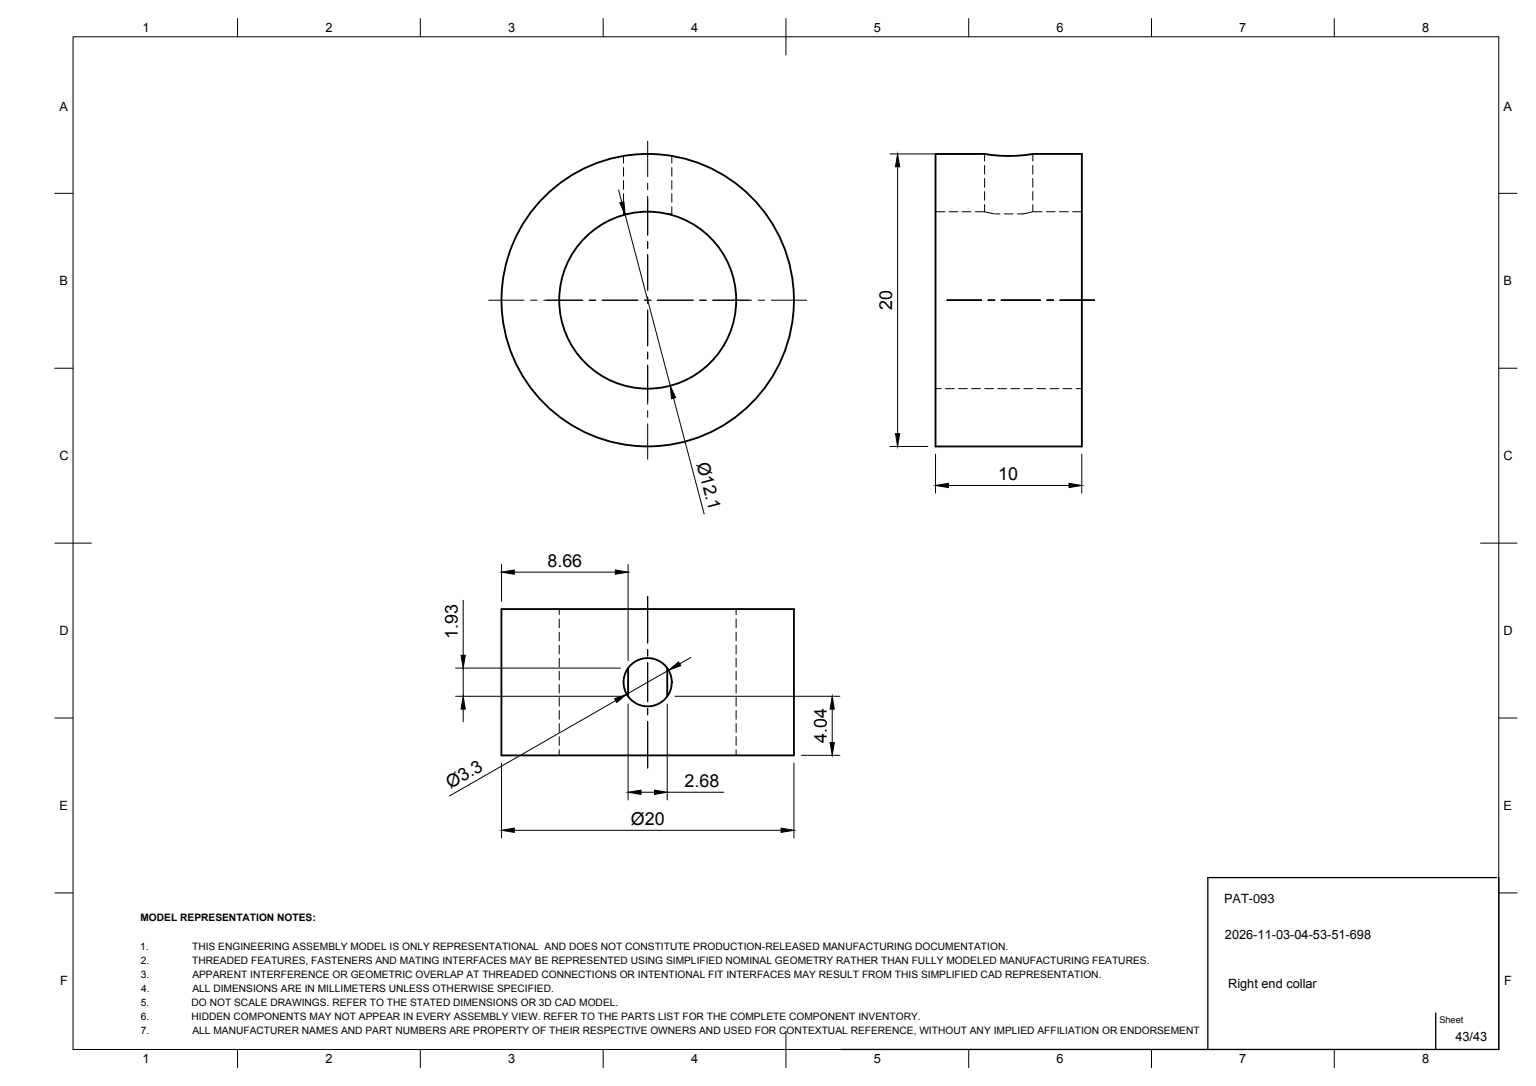
ISO-10303-21;
HEADER;
/* Generated by software containing ST-Developer
 * from STEP Tools, Inc. (www.steptools.com) 
 */

FILE_DESCRIPTION(
/* description */ ('Self-centering screw clamp'),
/* implementation_level */ '2;1');

FILE_NAME(
/* name */ 'Right end collar.step',
/* time_stamp */ '2026-10-28T03:25:31-07:00',
/* author */ (''),
/* organization */ (''),
/* preprocessor_version */ 'ST-DEVELOPER v20.2',
/* originating_system */ 'Autodesk Translation Framework v15.17.0.0',
/* authorisation */ '');

FILE_SCHEMA (('AUTOMOTIVE_DESIGN { 1 0 10303 214 3 1 1 }'));
ENDSEC;

DATA;
#10=MECHANICAL_DESIGN_GEOMETRIC_PRESENTATION_REPRESENTATION('',(#669),#16799);
#535=B_SPLINE_CURVE_WITH_KNOTS('',3,(#16377,#16378,#16379,#16380,#16381,
#16382,#16383,#16384),.UNSPECIFIED.,.F.,.F.,(4,2,2,4),(0.598759573717649,
0.624973342427789,0.687463163426141,0.749952984424493),.UNSPECIFIED.);
#536=B_SPLINE_CURVE_WITH_KNOTS('',3,(#16388,#16389,#16390,#16391,#16392,
#16393,#16394,#16395),.UNSPECIFIED.,.F.,.F.,(4,2,2,4),(0.249984328141498,
0.31247414913985,0.374963970138202,0.401177738848341),.UNSPECIFIED.);
#537=B_SPLINE_CURVE_WITH_KNOTS('',3,(#16396,#16397,#16398,#16399,#16400,
#16401,#16402,#16403),.UNSPECIFIED.,.F.,.F.,(4,2,2,4),(0.0987909174346529,
0.125004686144794,0.187494507143146,0.249984328141498),.UNSPECIFIED.);
#538=B_SPLINE_CURVE_WITH_KNOTS('',3,(#16404,#16405,#16406,#16407,#16408,
#16409,#16410,#16411),.UNSPECIFIED.,.F.,.F.,(4,2,2,4),(0.749952984424493,
0.812442805422846,0.874932626421198,0.901146395131338),.UNSPECIFIED.);
#539=B_SPLINE_CURVE_WITH_KNOTS('',3,(#16415,#16416,#16417,#16418,#16419,
#16420,#16421,#16422,#16423,#16424),.UNSPECIFIED.,.F.,.F.,(4,2,2,2,4),(0.,
0.0622766332261793,0.124553266452359,0.186828302721277,0.249103338990195),
 .UNSPECIFIED.);
#540=B_SPLINE_CURVE_WITH_KNOTS('',3,(#16426,#16427,#16428,#16429,#16430,
#16431,#16432,#16433,#16434,#16435),.UNSPECIFIED.,.F.,.F.,(4,2,2,2,4),(0.747310016970586,
0.809585053239505,0.871860089508423,0.934136722734602,0.996413355960782),
 .UNSPECIFIED.);
#541=B_SPLINE_CURVE_WITH_KNOTS('',3,(#16436,#16437,#16438,#16439,#16440,
#16441,#16442,#16443,#16444,#16445,#16446,#16447,#16448,#16449,#16450,#16451,
#16452,#16453),.UNSPECIFIED.,.F.,.F.,(4,2,2,2,2,2,2,2,4),(0.249103338990195,
0.311378375259114,0.373653411528032,0.435930044754212,0.498206677980391,
0.56048331120657,0.62275994443275,0.685034980701668,0.747310016970586),
 .UNSPECIFIED.);
#580=SHAPE_REPRESENTATION_RELATIONSHIP('SRR','None',#17058,#621);
#621=ADVANCED_BREP_SHAPE_REPRESENTATION('',(#716),#16796);
#669=STYLED_ITEM('',(#17340),#716);
#716=MANIFOLD_SOLID_BREP('Body1',#9121);
#1010=FACE_BOUND('',#2543,.T.);
#1011=FACE_BOUND('',#2545,.T.);
#1249=PLANE('',#10590);
#1250=PLANE('',#10594);
#1251=PLANE('',#10601);
#1252=PLANE('',#10602);
#1741=FACE_OUTER_BOUND('',#2537,.T.);
#1742=FACE_OUTER_BOUND('',#2538,.T.);
#1743=FACE_OUTER_BOUND('',#2539,.T.);
#1744=FACE_OUTER_BOUND('',#2540,.T.);
#1745=FACE_OUTER_BOUND('',#2541,.T.);
#1746=FACE_OUTER_BOUND('',#2542,.T.);
#1747=FACE_OUTER_BOUND('',#2544,.T.);
#2537=EDGE_LOOP('',(#8203,#8204));
#2538=EDGE_LOOP('',(#8205,#8206,#8207,#8208,#8209,#8210,#8211,#8212,#8213,
#8214,#8215));
#2539=EDGE_LOOP('',(#8216,#8217));
#2540=EDGE_LOOP('',(#8218,#8219,#8220,#8221,#8222,#8223,#8224,#8225,#8226,
#8227,#8228,#8229));
#2541=EDGE_LOOP('',(#8230,#8231,#8232,#8233,#8234,#8235,#8236,#8237,#8238));
#2542=EDGE_LOOP('',(#8239));
#2543=EDGE_LOOP('',(#8240));
#2544=EDGE_LOOP('',(#8241));
#2545=EDGE_LOOP('',(#8242));
#3098=LINE('',#16372,#3671);
#3099=LINE('',#16413,#3672);
#3100=LINE('',#16455,#3673);
#3101=LINE('',#16459,#3674);
#3102=LINE('',#16461,#3675);
#3103=LINE('',#16466,#3676);
#3104=LINE('',#16468,#3677);
#3671=VECTOR('',#13301,1.);
#3672=VECTOR('',#13308,0.164999999999999);
#3673=VECTOR('',#13311,1.);
#3674=VECTOR('',#13316,0.605);
#3675=VECTOR('',#13317,0.605);
#3676=VECTOR('',#13324,1.);
#3677=VECTOR('',#13325,1.);
#4215=CIRCLE('',#10591,0.164999999999999);
#4216=CIRCLE('',#10593,0.164999999999999);
#4217=CIRCLE('',#10596,0.605);
#4218=CIRCLE('',#10597,0.605);
#4219=CIRCLE('',#10599,1.);
#4220=CIRCLE('',#10600,1.);
#4927=VERTEX_POINT('',#16370);
#4928=VERTEX_POINT('',#16371);
#4929=VERTEX_POINT('',#16375);
#4930=VERTEX_POINT('',#16376);
#4931=VERTEX_POINT('',#16385);
#4932=VERTEX_POINT('',#16387);
#4933=VERTEX_POINT('',#16412);
#4934=VERTEX_POINT('',#16414);
#4935=VERTEX_POINT('',#16425);
#4936=VERTEX_POINT('',#16457);
#4937=VERTEX_POINT('',#16460);
#4938=VERTEX_POINT('',#16464);
#4939=VERTEX_POINT('',#16467);
#6026=EDGE_CURVE('',#4927,#4928,#3098,.T.);
#6027=EDGE_CURVE('',#4927,#4928,#4215,.T.);
#6028=EDGE_CURVE('',#4929,#4930,#535,.T.);
#6029=EDGE_CURVE('',#4931,#4929,#4216,.T.);
#6030=EDGE_CURVE('',#4932,#4931,#536,.T.);
#6031=EDGE_CURVE('',#4928,#4932,#537,.T.);
#6032=EDGE_CURVE('',#4930,#4927,#538,.T.);
#6033=EDGE_CURVE('',#4930,#4933,#3099,.T.);
#6034=EDGE_CURVE('',#4934,#4933,#539,.T.);
#6035=EDGE_CURVE('',#4935,#4934,#540,.T.);
#6036=EDGE_CURVE('',#4933,#4935,#541,.T.);
#6037=EDGE_CURVE('',#4931,#4929,#3100,.T.);
#6038=EDGE_CURVE('',#4936,#4936,#4217,.T.);
#6039=EDGE_CURVE('',#4936,#4932,#3101,.T.);
#6040=EDGE_CURVE('',#4930,#4937,#3102,.T.);
#6041=EDGE_CURVE('',#4937,#4937,#4218,.T.);
#6042=EDGE_CURVE('',#4938,#4938,#4219,.T.);
#6043=EDGE_CURVE('',#4938,#4935,#3103,.T.);
#6044=EDGE_CURVE('',#4933,#4939,#3104,.T.);
#6045=EDGE_CURVE('',#4939,#4939,#4220,.T.);
#8203=ORIENTED_EDGE('',*,*,#6026,.F.);
#8204=ORIENTED_EDGE('',*,*,#6027,.T.);
#8205=ORIENTED_EDGE('',*,*,#6028,.F.);
#8206=ORIENTED_EDGE('',*,*,#6029,.F.);
#8207=ORIENTED_EDGE('',*,*,#6030,.F.);
#8208=ORIENTED_EDGE('',*,*,#6031,.F.);
#8209=ORIENTED_EDGE('',*,*,#6027,.F.);
#8210=ORIENTED_EDGE('',*,*,#6032,.F.);
#8211=ORIENTED_EDGE('',*,*,#6033,.T.);
#8212=ORIENTED_EDGE('',*,*,#6034,.F.);
#8213=ORIENTED_EDGE('',*,*,#6035,.F.);
#8214=ORIENTED_EDGE('',*,*,#6036,.F.);
#8215=ORIENTED_EDGE('',*,*,#6033,.F.);
#8216=ORIENTED_EDGE('',*,*,#6037,.F.);
#8217=ORIENTED_EDGE('',*,*,#6029,.T.);
#8218=ORIENTED_EDGE('',*,*,#6038,.F.);
#8219=ORIENTED_EDGE('',*,*,#6039,.T.);
#8220=ORIENTED_EDGE('',*,*,#6030,.T.);
#8221=ORIENTED_EDGE('',*,*,#6037,.T.);
#8222=ORIENTED_EDGE('',*,*,#6028,.T.);
#8223=ORIENTED_EDGE('',*,*,#6040,.T.);
#8224=ORIENTED_EDGE('',*,*,#6041,.T.);
#8225=ORIENTED_EDGE('',*,*,#6040,.F.);
#8226=ORIENTED_EDGE('',*,*,#6032,.T.);
#8227=ORIENTED_EDGE('',*,*,#6026,.T.);
#8228=ORIENTED_EDGE('',*,*,#6031,.T.);
#8229=ORIENTED_EDGE('',*,*,#6039,.F.);
#8230=ORIENTED_EDGE('',*,*,#6042,.F.);
#8231=ORIENTED_EDGE('',*,*,#6043,.T.);
#8232=ORIENTED_EDGE('',*,*,#6035,.T.);
#8233=ORIENTED_EDGE('',*,*,#6034,.T.);
#8234=ORIENTED_EDGE('',*,*,#6044,.T.);
#8235=ORIENTED_EDGE('',*,*,#6045,.T.);
#8236=ORIENTED_EDGE('',*,*,#6044,.F.);
#8237=ORIENTED_EDGE('',*,*,#6036,.T.);
#8238=ORIENTED_EDGE('',*,*,#6043,.F.);
#8239=ORIENTED_EDGE('',*,*,#6042,.T.);
#8240=ORIENTED_EDGE('',*,*,#6038,.T.);
#8241=ORIENTED_EDGE('',*,*,#6045,.F.);
#8242=ORIENTED_EDGE('',*,*,#6041,.F.);
#8565=CYLINDRICAL_SURFACE('',#10592,0.164999999999999);
#8566=CYLINDRICAL_SURFACE('',#10595,0.605);
#8567=CYLINDRICAL_SURFACE('',#10598,1.);
#9039=ADVANCED_FACE('',(#1741),#1249,.T.);
#9040=ADVANCED_FACE('',(#1742),#8565,.F.);
#9041=ADVANCED_FACE('',(#1743),#1250,.T.);
#9042=ADVANCED_FACE('',(#1744),#8566,.F.);
#9043=ADVANCED_FACE('',(#1745),#8567,.T.);
#9044=ADVANCED_FACE('',(#1746,#1010),#1251,.T.);
#9045=ADVANCED_FACE('',(#1747,#1011),#1252,.F.);
#9121=CLOSED_SHELL('',(#9039,#9040,#9041,#9042,#9043,#9044,#9045));
#10589=AXIS2_PLACEMENT_3D('',#16368,#13297,#13298);
#10590=AXIS2_PLACEMENT_3D('',#16369,#13299,#13300);
#10591=AXIS2_PLACEMENT_3D('',#16373,#13302,#13303);
#10592=AXIS2_PLACEMENT_3D('',#16374,#13304,#13305);
#10593=AXIS2_PLACEMENT_3D('',#16386,#13306,#13307);
#10594=AXIS2_PLACEMENT_3D('',#16454,#13309,#13310);
#10595=AXIS2_PLACEMENT_3D('',#16456,#13312,#13313);
#10596=AXIS2_PLACEMENT_3D('',#16458,#13314,#13315);
#10597=AXIS2_PLACEMENT_3D('',#16462,#13318,#13319);
#10598=AXIS2_PLACEMENT_3D('',#16463,#13320,#13321);
#10599=AXIS2_PLACEMENT_3D('',#16465,#13322,#13323);
#10600=AXIS2_PLACEMENT_3D('',#16469,#13326,#13327);
#10601=AXIS2_PLACEMENT_3D('',#16470,#13328,#13329);
#10602=AXIS2_PLACEMENT_3D('',#16471,#13330,#13331);
#13297=DIRECTION('axis',(0.,0.,1.));
#13298=DIRECTION('refdir',(1.,0.,0.));
#13299=DIRECTION('center_axis',(0.,0.,1.));
#13300=DIRECTION('ref_axis',(1.,0.,0.));
#13301=DIRECTION('',(1.,0.,0.));
#13302=DIRECTION('center_axis',(0.,0.,1.));
#13303=DIRECTION('ref_axis',(1.,0.,0.));
#13304=DIRECTION('center_axis',(0.,0.,1.));
#13305=DIRECTION('ref_axis',(1.,0.,0.));
#13306=DIRECTION('center_axis',(0.,0.,1.));
#13307=DIRECTION('ref_axis',(1.,0.,0.));
#13308=DIRECTION('',(0.,0.,1.));
#13309=DIRECTION('center_axis',(0.,0.,1.));
#13310=DIRECTION('ref_axis',(1.,0.,0.));
#13311=DIRECTION('',(-1.,0.,0.));
#13312=DIRECTION('center_axis',(1.,0.,0.));
#13313=DIRECTION('ref_axis',(0.,0.,-1.));
#13314=DIRECTION('center_axis',(-1.,0.,0.));
#13315=DIRECTION('ref_axis',(0.,0.,-1.));
#13316=DIRECTION('',(-1.,0.,0.));
#13317=DIRECTION('',(-1.,0.,0.));
#13318=DIRECTION('center_axis',(-1.,0.,0.));
#13319=DIRECTION('ref_axis',(0.,0.,-1.));
#13320=DIRECTION('center_axis',(1.,0.,0.));
#13321=DIRECTION('ref_axis',(0.,0.,-1.));
#13322=DIRECTION('center_axis',(1.,0.,0.));
#13323=DIRECTION('ref_axis',(0.,0.,-1.));
#13324=DIRECTION('',(-1.,0.,0.));
#13325=DIRECTION('',(-1.,0.,0.));
#13326=DIRECTION('center_axis',(1.,0.,0.));
#13327=DIRECTION('ref_axis',(0.,0.,-1.));
#13328=DIRECTION('center_axis',(1.,0.,0.));
#13329=DIRECTION('ref_axis',(0.,0.,-1.));
#13330=DIRECTION('center_axis',(1.,0.,0.));
#13331=DIRECTION('ref_axis',(0.,0.,-1.));
#16368=CARTESIAN_POINT('',(0.,0.,0.));
#16369=CARTESIAN_POINT('Origin',(14.,0.,4.59));
#16370=CARTESIAN_POINT('',(13.9035634923901,-0.133884278389959,4.59));
#16371=CARTESIAN_POINT('',(14.0964365076099,-0.133884278389959,4.59));
#16372=CARTESIAN_POINT('',(13.5,-0.133884278389959,4.59));
#16373=CARTESIAN_POINT('Origin',(14.,0.,4.59));
#16374=CARTESIAN_POINT('Origin',(14.,0.,4.59));
#16375=CARTESIAN_POINT('',(13.9035634923901,0.133884278389959,4.59));
#16376=CARTESIAN_POINT('',(13.835,-8.64311690359451E-17,4.605));
#16377=CARTESIAN_POINT('Ctrl Pts',(13.9035634923901,0.133884278389959,4.59));
#16378=CARTESIAN_POINT('Ctrl Pts',(13.8962316423768,0.128603165341393,4.59119840340611));
#16379=CARTESIAN_POINT('Ctrl Pts',(13.8894472111884,0.122792448979943,4.59244064128815));
#16380=CARTESIAN_POINT('Ctrl Pts',(13.8687385941683,0.10208383195986,4.59651064111414));
#16381=CARTESIAN_POINT('Ctrl Pts',(13.8560565239921,0.0836002135946602,
4.59954409498317));
#16382=CARTESIAN_POINT('Ctrl Pts',(13.8391843843662,0.0429774150042655,
4.60381707438298));
#16383=CARTESIAN_POINT('Ctrl Pts',(13.835,0.0208299403327843,4.605));
#16384=CARTESIAN_POINT('Ctrl Pts',(13.835,1.94289029309402E-16,4.605));
#16385=CARTESIAN_POINT('',(14.0964365076099,0.133884278389959,4.59));
#16386=CARTESIAN_POINT('Origin',(14.,0.,4.59));
#16387=CARTESIAN_POINT('',(14.165,-1.96983309144393E-17,4.605));
#16388=CARTESIAN_POINT('Ctrl Pts',(14.165,3.46944695195361E-17,4.605));
#16389=CARTESIAN_POINT('Ctrl Pts',(14.165,0.0208299403327841,4.605));
#16390=CARTESIAN_POINT('Ctrl Pts',(14.1608156156338,0.0429774150042654,
4.60381707438298));
#16391=CARTESIAN_POINT('Ctrl Pts',(14.1439434760079,0.0836002135946602,
4.59954409498317));
#16392=CARTESIAN_POINT('Ctrl Pts',(14.1312614058317,0.10208383195986,4.59651064111414));
#16393=CARTESIAN_POINT('Ctrl Pts',(14.1105527888116,0.122792448979943,4.59244064128815));
#16394=CARTESIAN_POINT('Ctrl Pts',(14.1037683576232,0.128603165341394,4.59119840340611));
#16395=CARTESIAN_POINT('Ctrl Pts',(14.0964365076099,0.13388427838996,4.59));
#16396=CARTESIAN_POINT('Ctrl Pts',(14.0964365076099,-0.13388427838996,4.59));
#16397=CARTESIAN_POINT('Ctrl Pts',(14.1037683576232,-0.128603165341392,
4.59119840340611));
#16398=CARTESIAN_POINT('Ctrl Pts',(14.1105527888116,-0.122792448979944,
4.59244064128815));
#16399=CARTESIAN_POINT('Ctrl Pts',(14.1312614058317,-0.10208383195986,4.59651064111414));
#16400=CARTESIAN_POINT('Ctrl Pts',(14.1439434760079,-0.0836002135946602,
4.59954409498317));
#16401=CARTESIAN_POINT('Ctrl Pts',(14.1608156156338,-0.0429774150042654,
4.60381707438298));
#16402=CARTESIAN_POINT('Ctrl Pts',(14.165,-0.0208299403327839,4.605));
#16403=CARTESIAN_POINT('Ctrl Pts',(14.165,1.14491749414469E-16,4.605));
#16404=CARTESIAN_POINT('Ctrl Pts',(13.835,-1.52655665885959E-16,4.605));
#16405=CARTESIAN_POINT('Ctrl Pts',(13.835,-0.0208299403327842,4.605));
#16406=CARTESIAN_POINT('Ctrl Pts',(13.8391843843662,-0.0429774150042655,
4.60381707438298));
#16407=CARTESIAN_POINT('Ctrl Pts',(13.8560565239921,-0.0836002135946602,
4.59954409498317));
#16408=CARTESIAN_POINT('Ctrl Pts',(13.8687385941683,-0.10208383195986,4.59651064111414));
#16409=CARTESIAN_POINT('Ctrl Pts',(13.8894472111884,-0.122792448979943,
4.59244064128815));
#16410=CARTESIAN_POINT('Ctrl Pts',(13.8962316423768,-0.128603165341393,
4.59119840340611));
#16411=CARTESIAN_POINT('Ctrl Pts',(13.9035634923901,-0.133884278389959,
4.59));
#16412=CARTESIAN_POINT('',(13.835,-2.02066721859312E-17,5.));
#16413=CARTESIAN_POINT('',(13.835,-2.02066721859312E-17,4.59));
#16414=CARTESIAN_POINT('',(14.,-0.164999999999999,4.98629356684508));
#16415=CARTESIAN_POINT('Ctrl Pts',(14.,-0.164999999999999,4.98629356684508));
#16416=CARTESIAN_POINT('Ctrl Pts',(13.9792411222579,-0.164999999999999,
4.98629356684508));
#16417=CARTESIAN_POINT('Ctrl Pts',(13.9571250491954,-0.160843546393744,
4.98701673104451));
#16418=CARTESIAN_POINT('Ctrl Pts',(13.9164840215393,-0.143993021293681,
4.98961542163351));
#16419=CARTESIAN_POINT('Ctrl Pts',(13.8979557419361,-0.131300979727688,
4.99145196292459));
#16420=CARTESIAN_POINT('Ctrl Pts',(13.8686993953868,-0.102044633178354,
4.99488884996167));
#16421=CARTESIAN_POINT('Ctrl Pts',(13.8560070595837,-0.0835161924492572,
4.99671442041539));
#16422=CARTESIAN_POINT('Ctrl Pts',(13.8391563208071,-0.0428746115883117,
4.99928792543863));
#16423=CARTESIAN_POINT('Ctrl Pts',(13.835,-0.0207583454229728,5.));
#16424=CARTESIAN_POINT('Ctrl Pts',(13.835,4.85722573273506E-17,5.));
#16425=CARTESIAN_POINT('',(14.165,-3.34767643417387E-17,5.));
#16426=CARTESIAN_POINT('Ctrl Pts',(14.165,5.55111512312578E-17,5.));
#16427=CARTESIAN_POINT('Ctrl Pts',(14.165,-0.0207583454229728,5.));
#16428=CARTESIAN_POINT('Ctrl Pts',(14.1608436791929,-0.0428746115883117,
4.99928792543863));
#16429=CARTESIAN_POINT('Ctrl Pts',(14.1439929404163,-0.0835161924492572,
4.99671442041539));
#16430=CARTESIAN_POINT('Ctrl Pts',(14.1313006046132,-0.102044633178354,
4.99488884996167));
#16431=CARTESIAN_POINT('Ctrl Pts',(14.1020442580639,-0.131300979727688,
4.99145196292459));
#16432=CARTESIAN_POINT('Ctrl Pts',(14.0835159784607,-0.143993021293681,
4.98961542163351));
#16433=CARTESIAN_POINT('Ctrl Pts',(14.0428749508046,-0.160843546393744,
4.98701673104451));
#16434=CARTESIAN_POINT('Ctrl Pts',(14.0207588777421,-0.164999999999999,
4.98629356684508));
#16435=CARTESIAN_POINT('Ctrl Pts',(14.,-0.164999999999999,4.98629356684508));
#16436=CARTESIAN_POINT('Ctrl Pts',(13.835,-1.2490009027033E-16,5.));
#16437=CARTESIAN_POINT('Ctrl Pts',(13.835,0.0207583454229727,5.));
#16438=CARTESIAN_POINT('Ctrl Pts',(13.8391563208071,0.0428746115883117,
4.99928792543863));
#16439=CARTESIAN_POINT('Ctrl Pts',(13.8560070595837,0.0835161924492572,
4.99671442041539));
#16440=CARTESIAN_POINT('Ctrl Pts',(13.8686993953868,0.102044633178354,4.99488884996167));
#16441=CARTESIAN_POINT('Ctrl Pts',(13.8979557419361,0.131300979727688,4.99145196292459));
#16442=CARTESIAN_POINT('Ctrl Pts',(13.9164840215393,0.143993021293681,4.98961542163351));
#16443=CARTESIAN_POINT('Ctrl Pts',(13.9571250491954,0.160843546393744,4.98701673104451));
#16444=CARTESIAN_POINT('Ctrl Pts',(13.9792411222579,0.164999999999999,4.98629356684509));
#16445=CARTESIAN_POINT('Ctrl Pts',(14.0207588777421,0.164999999999999,4.98629356684509));
#16446=CARTESIAN_POINT('Ctrl Pts',(14.0428749508046,0.160843546393744,4.98701673104451));
#16447=CARTESIAN_POINT('Ctrl Pts',(14.0835159784607,0.143993021293681,4.98961542163351));
#16448=CARTESIAN_POINT('Ctrl Pts',(14.1020442580639,0.131300979727688,4.99145196292459));
#16449=CARTESIAN_POINT('Ctrl Pts',(14.1313006046132,0.102044633178354,4.99488884996167));
#16450=CARTESIAN_POINT('Ctrl Pts',(14.1439929404163,0.0835161924492573,
4.99671442041539));
#16451=CARTESIAN_POINT('Ctrl Pts',(14.1608436791929,0.0428746115883117,
4.99928792543863));
#16452=CARTESIAN_POINT('Ctrl Pts',(14.165,0.0207583454229729,5.));
#16453=CARTESIAN_POINT('Ctrl Pts',(14.165,1.45716771982052E-16,5.));
#16454=CARTESIAN_POINT('Origin',(14.,0.,4.59));
#16455=CARTESIAN_POINT('',(13.5,0.133884278389959,4.59));
#16456=CARTESIAN_POINT('Origin',(13.5,0.,4.));
#16457=CARTESIAN_POINT('',(14.5,-7.40911313484149E-17,4.605));
#16458=CARTESIAN_POINT('Origin',(14.5,0.,4.));
#16459=CARTESIAN_POINT('',(13.5,-7.40911313484149E-17,4.605));
#16460=CARTESIAN_POINT('',(13.5,-7.40911313484149E-17,4.605));
#16461=CARTESIAN_POINT('',(13.5,-7.40911313484149E-17,4.605));
#16462=CARTESIAN_POINT('Origin',(13.5,0.,4.));
#16463=CARTESIAN_POINT('Origin',(13.5,0.,4.));
#16464=CARTESIAN_POINT('',(14.5,-1.22464679914735E-16,5.));
#16465=CARTESIAN_POINT('Origin',(14.5,0.,4.));
#16466=CARTESIAN_POINT('',(13.5,-1.22464679914735E-16,5.));
#16467=CARTESIAN_POINT('',(13.5,-1.22464679914735E-16,5.));
#16468=CARTESIAN_POINT('',(13.5,-1.22464679914735E-16,5.));
#16469=CARTESIAN_POINT('Origin',(13.5,0.,4.));
#16470=CARTESIAN_POINT('Origin',(14.5,0.,4.));
#16471=CARTESIAN_POINT('Origin',(13.5,0.,4.));
#16747=UNCERTAINTY_MEASURE_WITH_UNIT(LENGTH_MEASURE(0.001),#16800,
'DISTANCE_ACCURACY_VALUE',
'Maximum model space distance between geometric entities at asserted c
onnectivities');
#16750=UNCERTAINTY_MEASURE_WITH_UNIT(LENGTH_MEASURE(0.001),#16800,
'DISTANCE_ACCURACY_VALUE',
'Maximum model space distance between geometric entities at asserted c
onnectivities');
#16796=(
GEOMETRIC_REPRESENTATION_CONTEXT(3)
GLOBAL_UNCERTAINTY_ASSIGNED_CONTEXT((#16747))
GLOBAL_UNIT_ASSIGNED_CONTEXT((#16800,#16802,#16803))
REPRESENTATION_CONTEXT('','3D')
);
#16799=(
GEOMETRIC_REPRESENTATION_CONTEXT(3)
GLOBAL_UNCERTAINTY_ASSIGNED_CONTEXT((#16750))
GLOBAL_UNIT_ASSIGNED_CONTEXT((#16800,#16802,#16803))
REPRESENTATION_CONTEXT('','3D')
);
#16800=(
LENGTH_UNIT()
NAMED_UNIT(*)
SI_UNIT(.CENTI.,.METRE.)
);
#16802=(
NAMED_UNIT(*)
PLANE_ANGLE_UNIT()
SI_UNIT($,.RADIAN.)
);
#16803=(
NAMED_UNIT(*)
SI_UNIT($,.STERADIAN.)
SOLID_ANGLE_UNIT()
);
#16849=SHAPE_DEFINITION_REPRESENTATION(#16904,#17058);
#16904=PRODUCT_DEFINITION_SHAPE('',$,#17107);
#17058=SHAPE_REPRESENTATION('',(#10589),#16796);
#17061=PRODUCT_DEFINITION_CONTEXT('part definition',#17207,'design');
#17107=PRODUCT_DEFINITION('Right end collar','Right end collar',#17155,
#17061);
#17155=PRODUCT_DEFINITION_FORMATION('',$,#17254);
#17207=APPLICATION_CONTEXT(
'Core Data for Automotive Mechanical Design Process');
#17208=PRODUCT_CONTEXT('part definition',#17207,'mechanical');
#17254=PRODUCT('Right end collar','Right end collar','Right end collar',
(#17208));
#17334=COLOUR_RGB('Off White',0.89,0.88,0.83);
#17335=FILL_AREA_STYLE_COLOUR('',#17334);
#17336=FILL_AREA_STYLE('',(#17335));
#17337=SURFACE_STYLE_FILL_AREA(#17336);
#17338=SURFACE_SIDE_STYLE('',(#17337));
#17339=SURFACE_STYLE_USAGE(.BOTH.,#17338);
#17340=PRESENTATION_STYLE_ASSIGNMENT((#17339));
ENDSEC;
END-ISO-10303-21;
